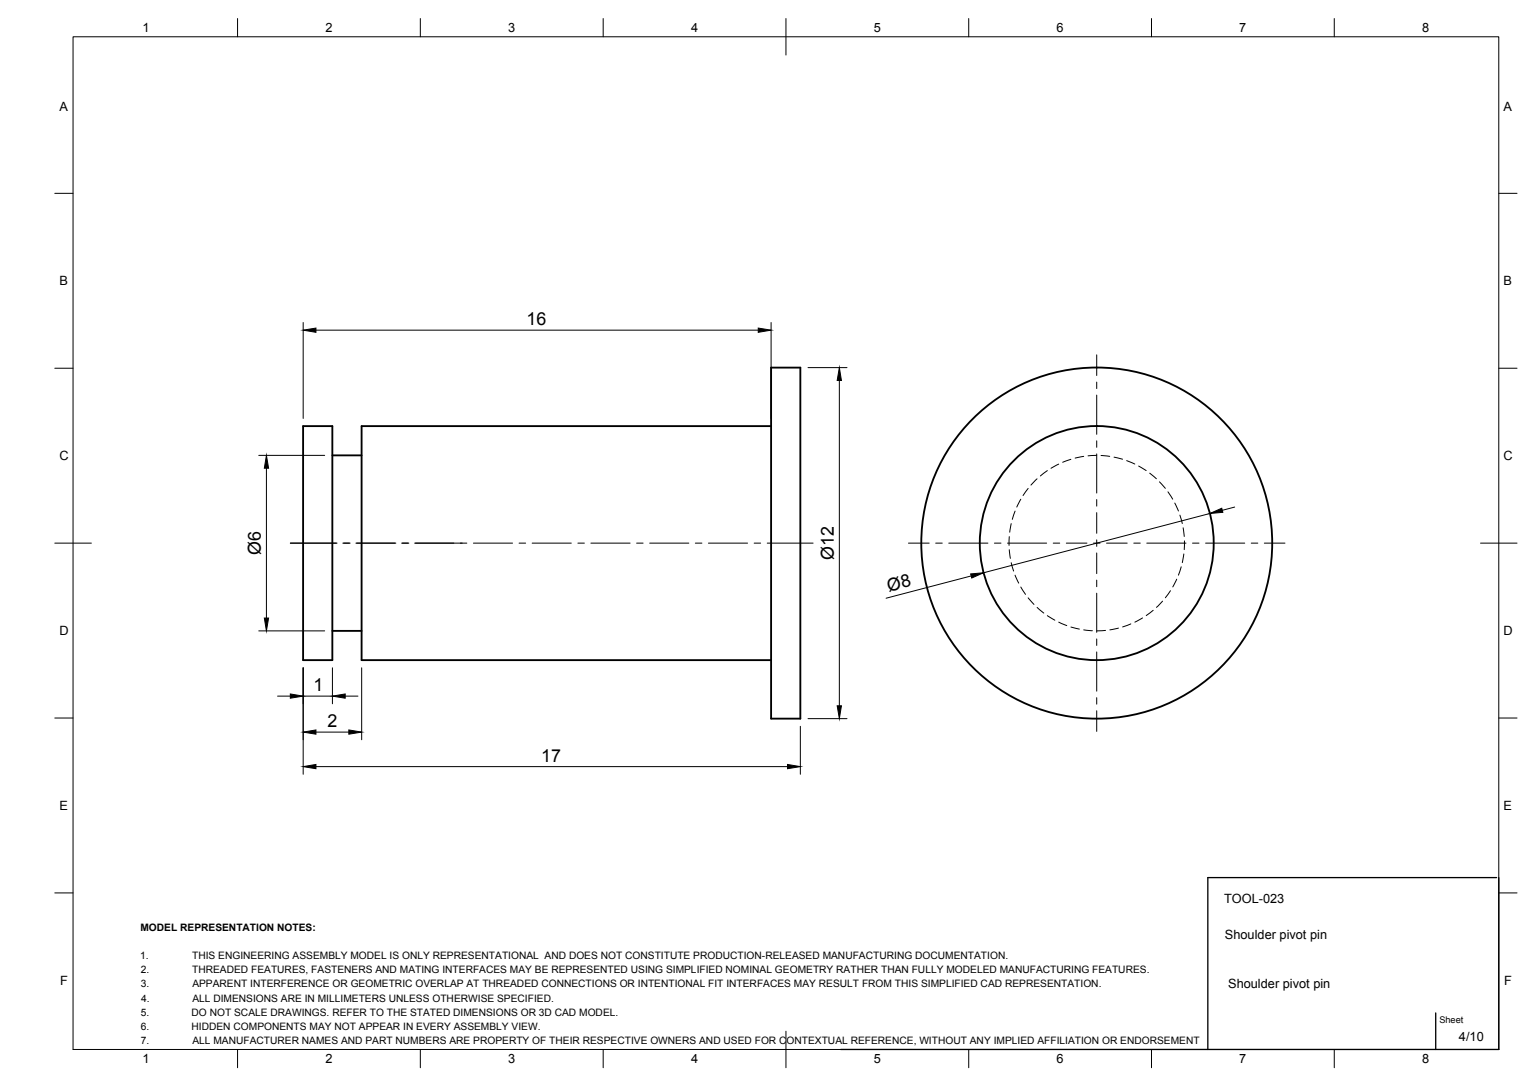
ISO-10303-21;
HEADER;
/* Generated by software containing ST-Developer
 * from STEP Tools, Inc. (www.steptools.com) 
 */

FILE_DESCRIPTION(
/* description */ (''),
/* implementation_level */ '2;1');

FILE_NAME(
/* name */ 'Shoulder pivot pin.step',
/* time_stamp */ '2026-11-10T05:40:20-08:00',
/* author */ (''),
/* organization */ (''),
/* preprocessor_version */ 'ST-DEVELOPER v20.2',
/* originating_system */ 'Autodesk Translation Framework v15.17.0.0',
/* authorisation */ '');

FILE_SCHEMA (('AUTOMOTIVE_DESIGN { 1 0 10303 214 3 1 1 }'));
ENDSEC;

DATA;
#10=MECHANICAL_DESIGN_GEOMETRIC_PRESENTATION_REPRESENTATION('',(#573),#18580);
#555=SHAPE_REPRESENTATION_RELATIONSHIP('SRR','None',#18625,#564);
#564=ADVANCED_BREP_SHAPE_REPRESENTATION('',(#582),#18571);
#573=STYLED_ITEM('',(#18684),#582);
#582=MANIFOLD_SOLID_BREP('Body1',#6545);
#596=FACE_BOUND('',#1207,.T.);
#597=FACE_BOUND('',#1209,.T.);
#598=FACE_BOUND('',#1212,.T.);
#673=PLANE('',#6696);
#674=PLANE('',#6698);
#675=PLANE('',#6702);
#676=PLANE('',#6707);
#677=PLANE('',#6709);
#823=FACE_OUTER_BOUND('',#1205,.T.);
#824=FACE_OUTER_BOUND('',#1206,.T.);
#825=FACE_OUTER_BOUND('',#1208,.T.);
#826=FACE_OUTER_BOUND('',#1210,.T.);
#827=FACE_OUTER_BOUND('',#1211,.T.);
#828=FACE_OUTER_BOUND('',#1213,.T.);
#829=FACE_OUTER_BOUND('',#1214,.T.);
#830=FACE_OUTER_BOUND('',#1215,.T.);
#831=FACE_OUTER_BOUND('',#1216,.T.);
#1205=EDGE_LOOP('',(#4286,#4287,#4288,#4289));
#1206=EDGE_LOOP('',(#4290));
#1207=EDGE_LOOP('',(#4291));
#1208=EDGE_LOOP('',(#4292));
#1209=EDGE_LOOP('',(#4293));
#1210=EDGE_LOOP('',(#4294,#4295,#4296,#4297));
#1211=EDGE_LOOP('',(#4298));
#1212=EDGE_LOOP('',(#4299));
#1213=EDGE_LOOP('',(#4300,#4301,#4302,#4303));
#1214=EDGE_LOOP('',(#4304));
#1215=EDGE_LOOP('',(#4305,#4306,#4307,#4308));
#1216=EDGE_LOOP('',(#4309));
#1672=LINE('',#8658,#2079);
#1673=LINE('',#8669,#2080);
#1674=LINE('',#8677,#2081);
#1675=LINE('',#8681,#2082);
#2079=VECTOR('',#7281,0.3);
#2080=VECTOR('',#7296,0.4);
#2081=VECTOR('',#7305,0.6);
#2082=VECTOR('',#7312,0.4);
#2433=CIRCLE('',#6694,0.3);
#2434=CIRCLE('',#6695,0.3);
#2435=CIRCLE('',#6697,0.4);
#2436=CIRCLE('',#6699,0.4);
#2437=CIRCLE('',#6701,0.4);
#2438=CIRCLE('',#6703,0.6);
#2439=CIRCLE('',#6704,0.4);
#2440=CIRCLE('',#6706,0.6);
#2629=VERTEX_POINT('',#8655);
#2630=VERTEX_POINT('',#8657);
#2631=VERTEX_POINT('',#8661);
#2632=VERTEX_POINT('',#8664);
#2633=VERTEX_POINT('',#8667);
#2634=VERTEX_POINT('',#8671);
#2635=VERTEX_POINT('',#8673);
#2636=VERTEX_POINT('',#8676);
#3266=EDGE_CURVE('',#2629,#2629,#2433,.T.);
#3267=EDGE_CURVE('',#2629,#2630,#1672,.T.);
#3268=EDGE_CURVE('',#2630,#2630,#2434,.T.);
#3269=EDGE_CURVE('',#2631,#2631,#2435,.T.);
#3270=EDGE_CURVE('',#2632,#2632,#2436,.T.);
#3271=EDGE_CURVE('',#2633,#2633,#2437,.T.);
#3272=EDGE_CURVE('',#2633,#2632,#1673,.T.);
#3273=EDGE_CURVE('',#2634,#2634,#2438,.T.);
#3274=EDGE_CURVE('',#2635,#2635,#2439,.T.);
#3275=EDGE_CURVE('',#2634,#2636,#1674,.T.);
#3276=EDGE_CURVE('',#2636,#2636,#2440,.T.);
#3277=EDGE_CURVE('',#2631,#2635,#1675,.T.);
#4286=ORIENTED_EDGE('',*,*,#3266,.T.);
#4287=ORIENTED_EDGE('',*,*,#3267,.T.);
#4288=ORIENTED_EDGE('',*,*,#3268,.F.);
#4289=ORIENTED_EDGE('',*,*,#3267,.F.);
#4290=ORIENTED_EDGE('',*,*,#3269,.F.);
#4291=ORIENTED_EDGE('',*,*,#3266,.F.);
#4292=ORIENTED_EDGE('',*,*,#3270,.F.);
#4293=ORIENTED_EDGE('',*,*,#3268,.T.);
#4294=ORIENTED_EDGE('',*,*,#3271,.F.);
#4295=ORIENTED_EDGE('',*,*,#3272,.T.);
#4296=ORIENTED_EDGE('',*,*,#3270,.T.);
#4297=ORIENTED_EDGE('',*,*,#3272,.F.);
#4298=ORIENTED_EDGE('',*,*,#3273,.T.);
#4299=ORIENTED_EDGE('',*,*,#3274,.F.);
#4300=ORIENTED_EDGE('',*,*,#3273,.F.);
#4301=ORIENTED_EDGE('',*,*,#3275,.T.);
#4302=ORIENTED_EDGE('',*,*,#3276,.T.);
#4303=ORIENTED_EDGE('',*,*,#3275,.F.);
#4304=ORIENTED_EDGE('',*,*,#3276,.F.);
#4305=ORIENTED_EDGE('',*,*,#3269,.T.);
#4306=ORIENTED_EDGE('',*,*,#3277,.T.);
#4307=ORIENTED_EDGE('',*,*,#3274,.T.);
#4308=ORIENTED_EDGE('',*,*,#3277,.F.);
#4309=ORIENTED_EDGE('',*,*,#3271,.T.);
#6039=CYLINDRICAL_SURFACE('',#6693,0.3);
#6040=CYLINDRICAL_SURFACE('',#6700,0.4);
#6041=CYLINDRICAL_SURFACE('',#6705,0.6);
#6042=CYLINDRICAL_SURFACE('',#6708,0.4);
#6195=ADVANCED_FACE('',(#823),#6039,.T.);
#6196=ADVANCED_FACE('',(#824,#596),#673,.F.);
#6197=ADVANCED_FACE('',(#825,#597),#674,.F.);
#6198=ADVANCED_FACE('',(#826),#6040,.T.);
#6199=ADVANCED_FACE('',(#827,#598),#675,.T.);
#6200=ADVANCED_FACE('',(#828),#6041,.T.);
#6201=ADVANCED_FACE('',(#829),#676,.F.);
#6202=ADVANCED_FACE('',(#830),#6042,.T.);
#6203=ADVANCED_FACE('',(#831),#677,.T.);
#6545=CLOSED_SHELL('',(#6195,#6196,#6197,#6198,#6199,#6200,#6201,#6202,
#6203));
#6692=AXIS2_PLACEMENT_3D('',#8653,#7275,#7276);
#6693=AXIS2_PLACEMENT_3D('',#8654,#7277,#7278);
#6694=AXIS2_PLACEMENT_3D('',#8656,#7279,#7280);
#6695=AXIS2_PLACEMENT_3D('',#8659,#7282,#7283);
#6696=AXIS2_PLACEMENT_3D('',#8660,#7284,#7285);
#6697=AXIS2_PLACEMENT_3D('',#8662,#7286,#7287);
#6698=AXIS2_PLACEMENT_3D('',#8663,#7288,#7289);
#6699=AXIS2_PLACEMENT_3D('',#8665,#7290,#7291);
#6700=AXIS2_PLACEMENT_3D('',#8666,#7292,#7293);
#6701=AXIS2_PLACEMENT_3D('',#8668,#7294,#7295);
#6702=AXIS2_PLACEMENT_3D('',#8670,#7297,#7298);
#6703=AXIS2_PLACEMENT_3D('',#8672,#7299,#7300);
#6704=AXIS2_PLACEMENT_3D('',#8674,#7301,#7302);
#6705=AXIS2_PLACEMENT_3D('',#8675,#7303,#7304);
#6706=AXIS2_PLACEMENT_3D('',#8678,#7306,#7307);
#6707=AXIS2_PLACEMENT_3D('',#8679,#7308,#7309);
#6708=AXIS2_PLACEMENT_3D('',#8680,#7310,#7311);
#6709=AXIS2_PLACEMENT_3D('',#8682,#7313,#7314);
#7275=DIRECTION('axis',(0.,0.,1.));
#7276=DIRECTION('refdir',(1.,0.,0.));
#7277=DIRECTION('center_axis',(0.,0.,1.));
#7278=DIRECTION('ref_axis',(1.,0.,0.));
#7279=DIRECTION('center_axis',(0.,0.,1.));
#7280=DIRECTION('ref_axis',(1.,0.,0.));
#7281=DIRECTION('',(0.,0.,1.));
#7282=DIRECTION('center_axis',(0.,0.,1.));
#7283=DIRECTION('ref_axis',(1.,0.,0.));
#7284=DIRECTION('center_axis',(0.,0.,-1.));
#7285=DIRECTION('ref_axis',(-1.,0.,0.));
#7286=DIRECTION('center_axis',(0.,0.,-1.));
#7287=DIRECTION('ref_axis',(1.,0.,0.));
#7288=DIRECTION('center_axis',(0.,0.,1.));
#7289=DIRECTION('ref_axis',(1.,0.,0.));
#7290=DIRECTION('center_axis',(0.,0.,1.));
#7291=DIRECTION('ref_axis',(1.,0.,0.));
#7292=DIRECTION('center_axis',(0.,0.,1.));
#7293=DIRECTION('ref_axis',(1.,0.,0.));
#7294=DIRECTION('center_axis',(0.,0.,1.));
#7295=DIRECTION('ref_axis',(1.,0.,0.));
#7296=DIRECTION('',(0.,0.,-1.));
#7297=DIRECTION('center_axis',(0.,0.,1.));
#7298=DIRECTION('ref_axis',(1.,0.,0.));
#7299=DIRECTION('center_axis',(0.,0.,1.));
#7300=DIRECTION('ref_axis',(1.,0.,0.));
#7301=DIRECTION('center_axis',(0.,0.,1.));
#7302=DIRECTION('ref_axis',(1.,0.,0.));
#7303=DIRECTION('center_axis',(0.,0.,1.));
#7304=DIRECTION('ref_axis',(1.,0.,0.));
#7305=DIRECTION('',(0.,0.,-1.));
#7306=DIRECTION('center_axis',(0.,0.,1.));
#7307=DIRECTION('ref_axis',(1.,0.,0.));
#7308=DIRECTION('center_axis',(0.,0.,1.));
#7309=DIRECTION('ref_axis',(1.,0.,0.));
#7310=DIRECTION('center_axis',(0.,0.,1.));
#7311=DIRECTION('ref_axis',(1.,0.,0.));
#7312=DIRECTION('',(0.,0.,-1.));
#7313=DIRECTION('center_axis',(0.,0.,1.));
#7314=DIRECTION('ref_axis',(1.,0.,0.));
#8653=CARTESIAN_POINT('',(0.,0.,0.));
#8654=CARTESIAN_POINT('Origin',(0.,0.,0.75));
#8655=CARTESIAN_POINT('',(-0.3,-3.67394039744206E-17,0.7));
#8656=CARTESIAN_POINT('Origin',(0.,0.,0.7));
#8657=CARTESIAN_POINT('',(-0.3,-3.67394039744206E-17,0.8));
#8658=CARTESIAN_POINT('',(-0.3,-3.67394039744206E-17,0.75));
#8659=CARTESIAN_POINT('Origin',(0.,0.,0.8));
#8660=CARTESIAN_POINT('Origin',(0.7,0.,0.7));
#8661=CARTESIAN_POINT('',(-0.4,4.89858719658941E-17,0.7));
#8662=CARTESIAN_POINT('Origin',(0.,0.,0.7));
#8663=CARTESIAN_POINT('Origin',(0.3,0.,0.8));
#8664=CARTESIAN_POINT('',(-0.4,-4.89858719658941E-17,0.8));
#8665=CARTESIAN_POINT('Origin',(0.,0.,0.8));
#8666=CARTESIAN_POINT('Origin',(0.,0.,-0.7));
#8667=CARTESIAN_POINT('',(-0.4,-4.89858719658941E-17,0.9));
#8668=CARTESIAN_POINT('Origin',(0.,0.,0.9));
#8669=CARTESIAN_POINT('',(-0.4,-4.89858719658941E-17,-0.7));
#8670=CARTESIAN_POINT('Origin',(0.,0.,-0.7));
#8671=CARTESIAN_POINT('',(-0.6,-7.34788079488412E-17,-0.7));
#8672=CARTESIAN_POINT('Origin',(0.,0.,-0.7));
#8673=CARTESIAN_POINT('',(-0.4,-4.89858719658941E-17,-0.7));
#8674=CARTESIAN_POINT('Origin',(0.,0.,-0.7));
#8675=CARTESIAN_POINT('Origin',(0.,0.,-0.8));
#8676=CARTESIAN_POINT('',(-0.6,-7.34788079488412E-17,-0.8));
#8677=CARTESIAN_POINT('',(-0.6,-7.34788079488412E-17,-0.8));
#8678=CARTESIAN_POINT('Origin',(0.,0.,-0.8));
#8679=CARTESIAN_POINT('Origin',(0.,0.,-0.8));
#8680=CARTESIAN_POINT('Origin',(0.,0.,-0.7));
#8681=CARTESIAN_POINT('',(-0.4,-4.89858719658941E-17,-0.7));
#8682=CARTESIAN_POINT('Origin',(0.,0.,0.9));
#18559=UNCERTAINTY_MEASURE_WITH_UNIT(LENGTH_MEASURE(0.001),#18581,
'DISTANCE_ACCURACY_VALUE',
'Maximum model space distance between geometric entities at asserted c
onnectivities');
#18568=UNCERTAINTY_MEASURE_WITH_UNIT(LENGTH_MEASURE(0.001),#18581,
'DISTANCE_ACCURACY_VALUE',
'Maximum model space distance between geometric entities at asserted c
onnectivities');
#18571=(
GEOMETRIC_REPRESENTATION_CONTEXT(3)
GLOBAL_UNCERTAINTY_ASSIGNED_CONTEXT((#18559))
GLOBAL_UNIT_ASSIGNED_CONTEXT((#18581,#18583,#18584))
REPRESENTATION_CONTEXT('','3D')
);
#18580=(
GEOMETRIC_REPRESENTATION_CONTEXT(3)
GLOBAL_UNCERTAINTY_ASSIGNED_CONTEXT((#18568))
GLOBAL_UNIT_ASSIGNED_CONTEXT((#18581,#18583,#18584))
REPRESENTATION_CONTEXT('','3D')
);
#18581=(
LENGTH_UNIT()
NAMED_UNIT(*)
SI_UNIT(.CENTI.,.METRE.)
);
#18583=(
NAMED_UNIT(*)
PLANE_ANGLE_UNIT()
SI_UNIT($,.RADIAN.)
);
#18584=(
NAMED_UNIT(*)
SI_UNIT($,.STERADIAN.)
SOLID_ANGLE_UNIT()
);
#18587=SHAPE_DEFINITION_REPRESENTATION(#18598,#18625);
#18598=PRODUCT_DEFINITION_SHAPE('',$,#18637);
#18625=SHAPE_REPRESENTATION('',(#6692),#18571);
#18634=PRODUCT_DEFINITION_CONTEXT('part definition',#18669,'design');
#18637=PRODUCT_DEFINITION('Shoulder pivot pin','Shoulder pivot pin',#18648,
#18634);
#18648=PRODUCT_DEFINITION_FORMATION('',$,#18673);
#18669=APPLICATION_CONTEXT(
'Core Data for Automotive Mechanical Design Process');
#18670=PRODUCT_CONTEXT('part definition',#18669,'mechanical');
#18673=PRODUCT('Shoulder pivot pin','Shoulder pivot pin',$,(#18670));
#18684=PRESENTATION_STYLE_ASSIGNMENT((#18692));
#18692=SURFACE_STYLE_USAGE(.BOTH.,#18700);
#18700=SURFACE_SIDE_STYLE('',(#18708));
#18708=SURFACE_STYLE_FILL_AREA(#18716);
#18716=FILL_AREA_STYLE('Pivot dark gray',(#18724));
#18724=FILL_AREA_STYLE_COLOUR('Pivot dark gray',#18732);
#18732=COLOUR_RGB('Pivot dark gray',0.27843137254902,0.309803921568627,
0.352941176470588);
ENDSEC;
END-ISO-10303-21;
